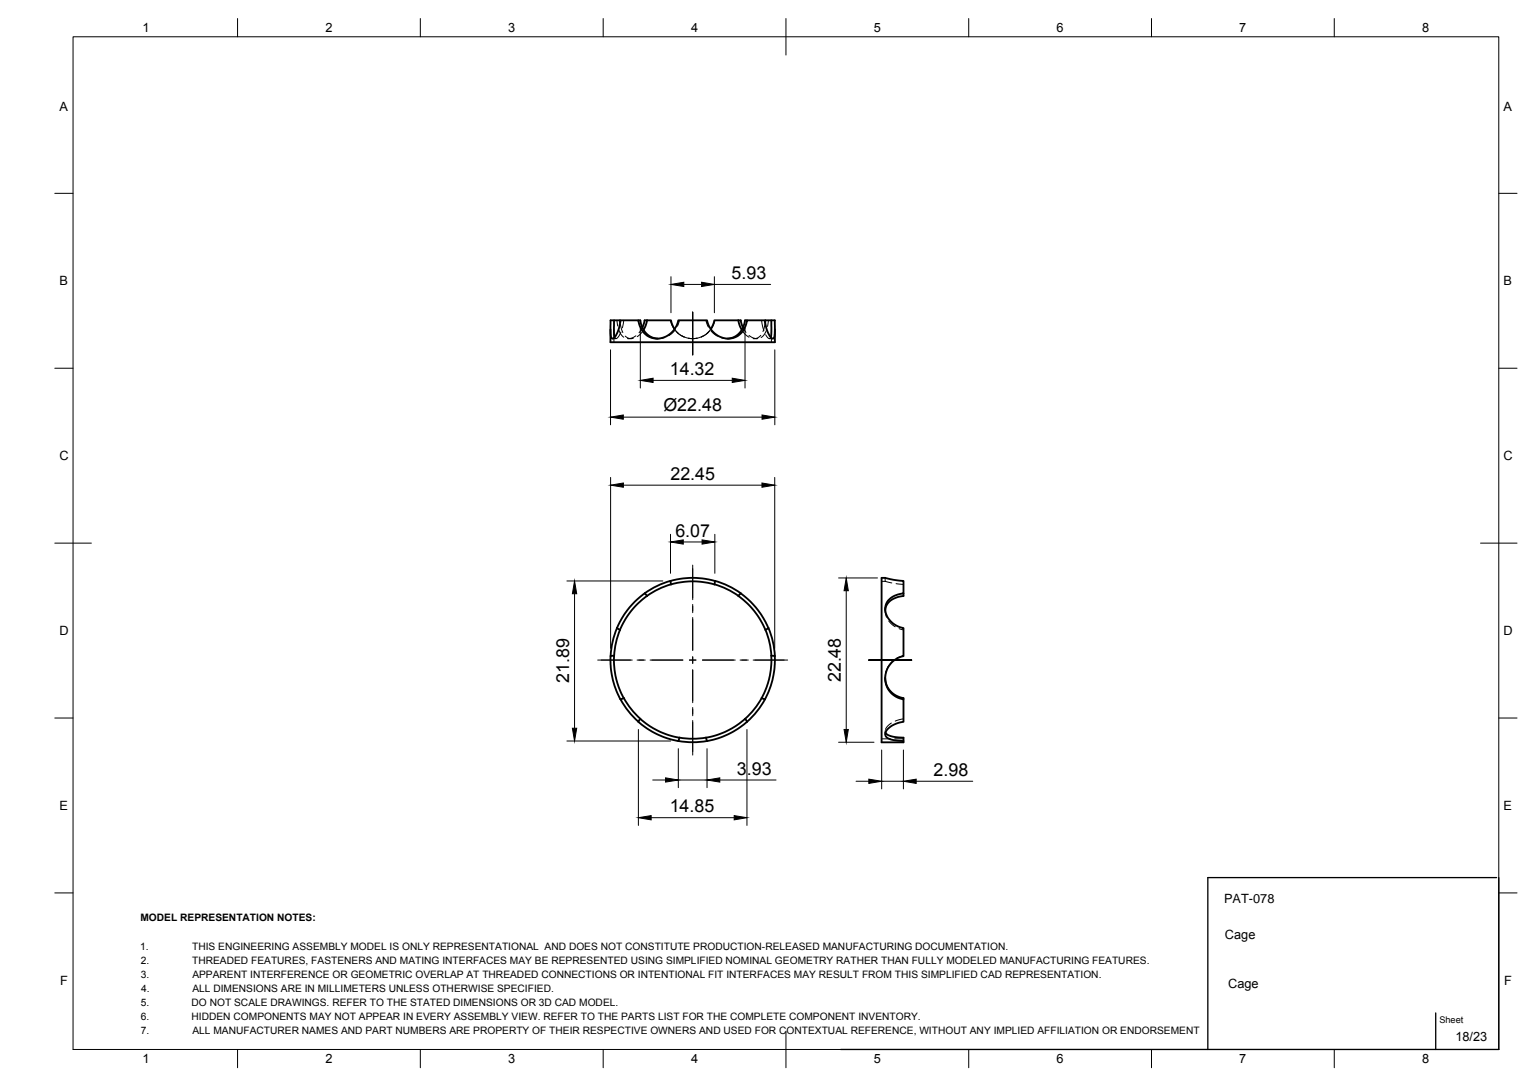
ISO-10303-21;
HEADER;
/* Generated by software containing ST-Developer
 * from STEP Tools, Inc. (www.steptools.com) 
 */

FILE_DESCRIPTION(
/* description */ ('Pedal-braked fixed caster'),
/* implementation_level */ '2;1');

FILE_NAME(
/* name */ 'Cage.step',
/* time_stamp */ '2026-10-28T03:26:52-07:00',
/* author */ (''),
/* organization */ (''),
/* preprocessor_version */ 'ST-DEVELOPER v20.2',
/* originating_system */ 'Autodesk Translation Framework v15.17.0.0',
/* authorisation */ '');

FILE_SCHEMA (('AUTOMOTIVE_DESIGN { 1 0 10303 214 3 1 1 }'));
ENDSEC;

DATA;
#10=MECHANICAL_DESIGN_GEOMETRIC_PRESENTATION_REPRESENTATION('',(#224),#5734);
#11=B_SPLINE_CURVE_WITH_KNOTS('',3,(#5151,#5152,#5153,#5154,#5155,#5156,
#5157,#5158,#5159,#5160,#5161,#5162,#5163,#5164,#5165,#5166,#5167,#5168,
#5169,#5170,#5171,#5172),.UNSPECIFIED.,.F.,.F.,(4,2,2,2,2,2,2,2,2,2,4),
(0.0591825211272536,0.157966726598481,0.236950089897721,0.315933453196962,
0.391576304923761,0.46721915665056,0.54286200837736,0.618504860104159,0.697488223403399,
0.77647158670264,0.875255792173867),.UNSPECIFIED.);
#12=B_SPLINE_CURVE_WITH_KNOTS('',3,(#5176,#5177,#5178,#5179,#5180,#5181,
#5182,#5183,#5184,#5185,#5186,#5187,#5188,#5189,#5190,#5191,#5192,#5193,
#5194,#5195,#5196,#5197),.UNSPECIFIED.,.F.,.F.,(4,2,2,2,2,2,2,2,2,2,4),
(0.0581119756758434,0.106553146291161,0.213106292582322,0.30849933801665,
0.386091982889075,0.4636846277615,0.541277272633925,0.61886991750635,0.714262962940678,
0.820816109231839,0.869257279847157),.UNSPECIFIED.);
#13=B_SPLINE_CURVE_WITH_KNOTS('',3,(#5203,#5204,#5205,#5206,#5207,#5208,
#5209,#5210,#5211,#5212,#5213,#5214,#5215,#5216,#5217,#5218,#5219,#5220,
#5221,#5222,#5223,#5224),.UNSPECIFIED.,.F.,.F.,(4,2,2,2,2,2,2,2,2,2,4),
(0.0581119756758434,0.106553146291161,0.213106292582322,0.30849933801665,
0.386091982889075,0.4636846277615,0.541277272633925,0.61886991750635,0.714262962940679,
0.820816109231839,0.869257279847157),.UNSPECIFIED.);
#14=B_SPLINE_CURVE_WITH_KNOTS('',3,(#5228,#5229,#5230,#5231,#5232,#5233,
#5234,#5235,#5236,#5237,#5238,#5239,#5240,#5241,#5242,#5243,#5244,#5245,
#5246,#5247,#5248,#5249),.UNSPECIFIED.,.F.,.F.,(4,2,2,2,2,2,2,2,2,2,4),
(0.0581119756758433,0.106553146291161,0.213106292582322,0.308499338016649,
0.386091982889075,0.4636846277615,0.541277272633925,0.61886991750635,0.714262962940678,
0.820816109231839,0.869257279847157),.UNSPECIFIED.);
#15=B_SPLINE_CURVE_WITH_KNOTS('',3,(#5258,#5259,#5260,#5261,#5262,#5263,
#5264,#5265,#5266,#5267,#5268,#5269,#5270,#5271,#5272,#5273,#5274,#5275,
#5276,#5277,#5278,#5279),.UNSPECIFIED.,.F.,.F.,(4,2,2,2,2,2,2,2,2,2,4),
(0.0581119756758433,0.106553146291161,0.213106292582322,0.30849933801665,
0.386091982889075,0.4636846277615,0.541277272633925,0.61886991750635,0.714262962940678,
0.820816109231839,0.869257279847157),.UNSPECIFIED.);
#16=B_SPLINE_CURVE_WITH_KNOTS('',3,(#5283,#5284,#5285,#5286,#5287,#5288,
#5289,#5290,#5291,#5292,#5293,#5294,#5295,#5296,#5297,#5298,#5299,#5300,
#5301,#5302,#5303,#5304),.UNSPECIFIED.,.F.,.F.,(4,2,2,2,2,2,2,2,2,2,4),
(0.0581119756758434,0.106553146291161,0.213106292582322,0.30849933801665,
0.386091982889075,0.4636846277615,0.541277272633925,0.61886991750635,0.714262962940678,
0.820816109231839,0.869257279847157),.UNSPECIFIED.);
#17=B_SPLINE_CURVE_WITH_KNOTS('',3,(#5308,#5309,#5310,#5311,#5312,#5313,
#5314,#5315,#5316,#5317,#5318,#5319,#5320,#5321,#5322,#5323,#5324,#5325,
#5326,#5327,#5328,#5329),.UNSPECIFIED.,.F.,.F.,(4,2,2,2,2,2,2,2,2,2,4),
(0.0581119756758434,0.106553146291161,0.213106292582322,0.30849933801665,
0.386091982889075,0.4636846277615,0.541277272633925,0.61886991750635,0.714262962940678,
0.820816109231839,0.869257279847157),.UNSPECIFIED.);
#18=B_SPLINE_CURVE_WITH_KNOTS('',3,(#5333,#5334,#5335,#5336,#5337,#5338,
#5339,#5340,#5341,#5342,#5343,#5344,#5345,#5346,#5347,#5348,#5349,#5350,
#5351,#5352,#5353,#5354),.UNSPECIFIED.,.F.,.F.,(4,2,2,2,2,2,2,2,2,2,4),
(0.0581119756758433,0.106553146291161,0.213106292582322,0.30849933801665,
0.386091982889075,0.4636846277615,0.541277272633925,0.61886991750635,0.714262962940678,
0.820816109231839,0.869257279847157),.UNSPECIFIED.);
#19=B_SPLINE_CURVE_WITH_KNOTS('',3,(#5362,#5363,#5364,#5365,#5366,#5367,
#5368,#5369,#5370,#5371,#5372,#5373,#5374,#5375,#5376,#5377,#5378,#5379,
#5380,#5381,#5382,#5383),.UNSPECIFIED.,.F.,.F.,(4,2,2,2,2,2,2,2,2,2,4),
(0.0591825211272536,0.157966726598481,0.236950089897721,0.315933453196962,
0.391576304923761,0.467219156650561,0.54286200837736,0.618504860104159,
0.697488223403399,0.77647158670264,0.875255792173867),.UNSPECIFIED.);
#20=B_SPLINE_CURVE_WITH_KNOTS('',3,(#5391,#5392,#5393,#5394,#5395,#5396,
#5397,#5398,#5399,#5400,#5401,#5402,#5403,#5404,#5405,#5406,#5407,#5408,
#5409,#5410,#5411,#5412),.UNSPECIFIED.,.F.,.F.,(4,2,2,2,2,2,2,2,2,2,4),
(0.0591825211272536,0.157966726598481,0.236950089897722,0.315933453196962,
0.391576304923761,0.467219156650561,0.54286200837736,0.618504860104159,
0.697488223403399,0.77647158670264,0.875255792173867),.UNSPECIFIED.);
#21=B_SPLINE_CURVE_WITH_KNOTS('',3,(#5422,#5423,#5424,#5425,#5426,#5427,
#5428,#5429,#5430,#5431,#5432,#5433,#5434,#5435,#5436,#5437,#5438,#5439,
#5440,#5441,#5442,#5443),.UNSPECIFIED.,.F.,.F.,(4,2,2,2,2,2,2,2,2,2,4),
(0.0591825211272536,0.157966726598481,0.236950089897721,0.315933453196962,
0.391576304923761,0.46721915665056,0.54286200837736,0.618504860104159,0.697488223403399,
0.77647158670264,0.875255792173867),.UNSPECIFIED.);
#22=B_SPLINE_CURVE_WITH_KNOTS('',3,(#5451,#5452,#5453,#5454,#5455,#5456,
#5457,#5458,#5459,#5460,#5461,#5462,#5463,#5464,#5465,#5466,#5467,#5468,
#5469,#5470,#5471,#5472),.UNSPECIFIED.,.F.,.F.,(4,2,2,2,2,2,2,2,2,2,4),
(0.0591825211272536,0.157966726598481,0.236950089897721,0.315933453196962,
0.391576304923761,0.46721915665056,0.542862008377359,0.618504860104159,
0.697488223403399,0.776471586702639,0.875255792173867),.UNSPECIFIED.);
#23=B_SPLINE_CURVE_WITH_KNOTS('',3,(#5480,#5481,#5482,#5483,#5484,#5485,
#5486,#5487,#5488,#5489,#5490,#5491,#5492,#5493,#5494,#5495,#5496,#5497,
#5498,#5499,#5500,#5501),.UNSPECIFIED.,.F.,.F.,(4,2,2,2,2,2,2,2,2,2,4),
(0.0591825211272536,0.157966726598481,0.236950089897721,0.315933453196962,
0.391576304923761,0.46721915665056,0.54286200837736,0.618504860104159,0.697488223403399,
0.77647158670264,0.875255792173867),.UNSPECIFIED.);
#24=B_SPLINE_CURVE_WITH_KNOTS('',3,(#5510,#5511,#5512,#5513,#5514,#5515,
#5516,#5517,#5518,#5519,#5520,#5521,#5522,#5523,#5524,#5525,#5526,#5527,
#5528,#5529,#5530,#5531),.UNSPECIFIED.,.F.,.F.,(4,2,2,2,2,2,2,2,2,2,4),
(0.0591825211272536,0.157966726598481,0.236950089897721,0.315933453196962,
0.391576304923761,0.46721915665056,0.542862008377359,0.618504860104159,
0.697488223403399,0.776471586702639,0.875255792173867),.UNSPECIFIED.);
#32=SPHERICAL_SURFACE('',#3444,0.309556);
#33=SPHERICAL_SURFACE('',#3460,0.309556);
#34=SPHERICAL_SURFACE('',#3465,0.309556);
#35=SPHERICAL_SURFACE('',#3471,0.309556);
#36=SPHERICAL_SURFACE('',#3476,0.309556);
#37=SPHERICAL_SURFACE('',#3481,0.309556);
#38=SPHERICAL_SURFACE('',#3489,0.309556);
#184=SHAPE_REPRESENTATION_RELATIONSHIP('SRR','None',#5824,#201);
#201=ADVANCED_BREP_SHAPE_REPRESENTATION('',(#247),#5728);
#224=STYLED_ITEM('',(#5984),#247);
#247=MANIFOLD_SOLID_BREP('Continuous crown cage',#3006);
#284=CYLINDRICAL_SURFACE('',#3447,1.123812);
#285=CYLINDRICAL_SURFACE('',#3483,1.076188);
#331=FACE_BOUND('',#837,.T.);
#426=CIRCLE('',#3445,0.303778037777585);
#427=CIRCLE('',#3446,0.303778037777585);
#428=CIRCLE('',#3448,1.123812);
#429=CIRCLE('',#3449,1.123812);
#430=CIRCLE('',#3450,1.123812);
#431=CIRCLE('',#3451,1.123812);
#432=CIRCLE('',#3452,1.123812);
#433=CIRCLE('',#3453,1.123812);
#434=CIRCLE('',#3454,1.123812);
#435=CIRCLE('',#3455,1.123812);
#436=CIRCLE('',#3456,1.123812);
#437=CIRCLE('',#3458,1.076188);
#438=CIRCLE('',#3459,0.303778037777585);
#439=CIRCLE('',#3461,0.303778037777585);
#440=CIRCLE('',#3463,1.076188);
#441=CIRCLE('',#3464,0.303778037777585);
#442=CIRCLE('',#3466,0.303778037777585);
#443=CIRCLE('',#3468,1.076188);
#444=CIRCLE('',#3469,1.076188);
#445=CIRCLE('',#3470,0.303778037777585);
#446=CIRCLE('',#3472,0.303778037777585);
#447=CIRCLE('',#3474,1.076188);
#448=CIRCLE('',#3475,0.303778037777585);
#449=CIRCLE('',#3477,0.303778037777585);
#450=CIRCLE('',#3479,1.076188);
#451=CIRCLE('',#3480,0.303778037777585);
#452=CIRCLE('',#3482,0.303778037777585);
#453=CIRCLE('',#3484,1.076188);
#454=CIRCLE('',#3485,1.076188);
#455=CIRCLE('',#3486,1.076188);
#456=CIRCLE('',#3488,0.303778037777585);
#457=CIRCLE('',#3490,0.303778037777585);
#607=FACE_OUTER_BOUND('',#821,.T.);
#608=FACE_OUTER_BOUND('',#822,.T.);
#609=FACE_OUTER_BOUND('',#823,.T.);
#610=FACE_OUTER_BOUND('',#824,.T.);
#611=FACE_OUTER_BOUND('',#825,.T.);
#612=FACE_OUTER_BOUND('',#826,.T.);
#613=FACE_OUTER_BOUND('',#827,.T.);
#614=FACE_OUTER_BOUND('',#828,.T.);
#615=FACE_OUTER_BOUND('',#829,.T.);
#616=FACE_OUTER_BOUND('',#830,.T.);
#617=FACE_OUTER_BOUND('',#831,.T.);
#618=FACE_OUTER_BOUND('',#832,.T.);
#619=FACE_OUTER_BOUND('',#833,.T.);
#620=FACE_OUTER_BOUND('',#834,.T.);
#621=FACE_OUTER_BOUND('',#835,.T.);
#622=FACE_OUTER_BOUND('',#836,.T.);
#623=FACE_OUTER_BOUND('',#838,.T.);
#821=EDGE_LOOP('',(#2484,#2485,#2486,#2487));
#822=EDGE_LOOP('',(#2488,#2489,#2490,#2491,#2492,#2493,#2494,#2495,#2496,
#2497,#2498,#2499,#2500,#2501,#2502,#2503,#2504,#2505));
#823=EDGE_LOOP('',(#2506,#2507,#2508,#2509));
#824=EDGE_LOOP('',(#2510,#2511,#2512,#2513));
#825=EDGE_LOOP('',(#2514,#2515,#2516,#2517));
#826=EDGE_LOOP('',(#2518,#2519,#2520,#2521));
#827=EDGE_LOOP('',(#2522,#2523,#2524,#2525,#2526,#2527));
#828=EDGE_LOOP('',(#2528,#2529,#2530,#2531));
#829=EDGE_LOOP('',(#2532,#2533,#2534,#2535));
#830=EDGE_LOOP('',(#2536,#2537,#2538,#2539));
#831=EDGE_LOOP('',(#2540,#2541,#2542,#2543));
#832=EDGE_LOOP('',(#2544,#2545,#2546,#2547));
#833=EDGE_LOOP('',(#2548,#2549,#2550,#2551,#2552,#2553,#2554,#2555,#2556,
#2557,#2558,#2559,#2560,#2561,#2562,#2563,#2564,#2565));
#834=EDGE_LOOP('',(#2566,#2567,#2568,#2569));
#835=EDGE_LOOP('',(#2570,#2571,#2572,#2573));
#836=EDGE_LOOP('',(#2574));
#837=EDGE_LOOP('',(#2575));
#838=EDGE_LOOP('',(#2576,#2577,#2578,#2579));
#1045=LINE('',#5253,#1257);
#1046=LINE('',#5506,#1258);
#1257=VECTOR('',#4231,1.123812);
#1258=VECTOR('',#4300,1.076188);
#1488=VERTEX_POINT('',#5149);
#1489=VERTEX_POINT('',#5150);
#1490=VERTEX_POINT('',#5173);
#1491=VERTEX_POINT('',#5175);
#1492=VERTEX_POINT('',#5200);
#1493=VERTEX_POINT('',#5202);
#1494=VERTEX_POINT('',#5225);
#1495=VERTEX_POINT('',#5227);
#1496=VERTEX_POINT('',#5250);
#1497=VERTEX_POINT('',#5252);
#1498=VERTEX_POINT('',#5255);
#1499=VERTEX_POINT('',#5257);
#1500=VERTEX_POINT('',#5280);
#1501=VERTEX_POINT('',#5282);
#1502=VERTEX_POINT('',#5305);
#1503=VERTEX_POINT('',#5307);
#1504=VERTEX_POINT('',#5330);
#1505=VERTEX_POINT('',#5332);
#1506=VERTEX_POINT('',#5357);
#1507=VERTEX_POINT('',#5361);
#1508=VERTEX_POINT('',#5386);
#1509=VERTEX_POINT('',#5390);
#1510=VERTEX_POINT('',#5415);
#1511=VERTEX_POINT('',#5417);
#1512=VERTEX_POINT('',#5421);
#1513=VERTEX_POINT('',#5446);
#1514=VERTEX_POINT('',#5450);
#1515=VERTEX_POINT('',#5475);
#1516=VERTEX_POINT('',#5479);
#1517=VERTEX_POINT('',#5504);
#1518=VERTEX_POINT('',#5507);
#1519=VERTEX_POINT('',#5509);
#1832=EDGE_CURVE('',#1488,#1489,#11,.T.);
#1833=EDGE_CURVE('',#1490,#1488,#426,.T.);
#1834=EDGE_CURVE('',#1491,#1490,#12,.T.);
#1835=EDGE_CURVE('',#1489,#1491,#427,.T.);
#1836=EDGE_CURVE('',#1492,#1490,#428,.T.);
#1837=EDGE_CURVE('',#1492,#1493,#13,.T.);
#1838=EDGE_CURVE('',#1494,#1493,#429,.T.);
#1839=EDGE_CURVE('',#1494,#1495,#14,.T.);
#1840=EDGE_CURVE('',#1496,#1495,#430,.T.);
#1841=EDGE_CURVE('',#1496,#1497,#1045,.T.);
#1842=EDGE_CURVE('',#1497,#1497,#431,.T.);
#1843=EDGE_CURVE('',#1498,#1496,#432,.T.);
#1844=EDGE_CURVE('',#1498,#1499,#15,.T.);
#1845=EDGE_CURVE('',#1500,#1499,#433,.T.);
#1846=EDGE_CURVE('',#1500,#1501,#16,.T.);
#1847=EDGE_CURVE('',#1502,#1501,#434,.T.);
#1848=EDGE_CURVE('',#1502,#1503,#17,.T.);
#1849=EDGE_CURVE('',#1504,#1503,#435,.T.);
#1850=EDGE_CURVE('',#1504,#1505,#18,.T.);
#1851=EDGE_CURVE('',#1491,#1505,#436,.T.);
#1852=EDGE_CURVE('',#1488,#1506,#437,.T.);
#1853=EDGE_CURVE('',#1506,#1492,#438,.T.);
#1854=EDGE_CURVE('',#1507,#1506,#19,.T.);
#1855=EDGE_CURVE('',#1493,#1507,#439,.T.);
#1856=EDGE_CURVE('',#1507,#1508,#440,.T.);
#1857=EDGE_CURVE('',#1508,#1494,#441,.T.);
#1858=EDGE_CURVE('',#1509,#1508,#20,.T.);
#1859=EDGE_CURVE('',#1495,#1509,#442,.T.);
#1860=EDGE_CURVE('',#1509,#1510,#443,.T.);
#1861=EDGE_CURVE('',#1510,#1511,#444,.T.);
#1862=EDGE_CURVE('',#1511,#1498,#445,.T.);
#1863=EDGE_CURVE('',#1512,#1511,#21,.T.);
#1864=EDGE_CURVE('',#1499,#1512,#446,.T.);
#1865=EDGE_CURVE('',#1512,#1513,#447,.T.);
#1866=EDGE_CURVE('',#1513,#1500,#448,.T.);
#1867=EDGE_CURVE('',#1514,#1513,#22,.T.);
#1868=EDGE_CURVE('',#1501,#1514,#449,.T.);
#1869=EDGE_CURVE('',#1514,#1515,#450,.T.);
#1870=EDGE_CURVE('',#1515,#1502,#451,.T.);
#1871=EDGE_CURVE('',#1516,#1515,#23,.T.);
#1872=EDGE_CURVE('',#1503,#1516,#452,.T.);
#1873=EDGE_CURVE('',#1517,#1517,#453,.T.);
#1874=EDGE_CURVE('',#1517,#1510,#1046,.T.);
#1875=EDGE_CURVE('',#1518,#1489,#454,.T.);
#1876=EDGE_CURVE('',#1518,#1519,#24,.T.);
#1877=EDGE_CURVE('',#1516,#1519,#455,.T.);
#1878=EDGE_CURVE('',#1505,#1518,#456,.T.);
#1879=EDGE_CURVE('',#1519,#1504,#457,.T.);
#2484=ORIENTED_EDGE('',*,*,#1832,.F.);
#2485=ORIENTED_EDGE('',*,*,#1833,.F.);
#2486=ORIENTED_EDGE('',*,*,#1834,.F.);
#2487=ORIENTED_EDGE('',*,*,#1835,.F.);
#2488=ORIENTED_EDGE('',*,*,#1834,.T.);
#2489=ORIENTED_EDGE('',*,*,#1836,.F.);
#2490=ORIENTED_EDGE('',*,*,#1837,.T.);
#2491=ORIENTED_EDGE('',*,*,#1838,.F.);
#2492=ORIENTED_EDGE('',*,*,#1839,.T.);
#2493=ORIENTED_EDGE('',*,*,#1840,.F.);
#2494=ORIENTED_EDGE('',*,*,#1841,.T.);
#2495=ORIENTED_EDGE('',*,*,#1842,.F.);
#2496=ORIENTED_EDGE('',*,*,#1841,.F.);
#2497=ORIENTED_EDGE('',*,*,#1843,.F.);
#2498=ORIENTED_EDGE('',*,*,#1844,.T.);
#2499=ORIENTED_EDGE('',*,*,#1845,.F.);
#2500=ORIENTED_EDGE('',*,*,#1846,.T.);
#2501=ORIENTED_EDGE('',*,*,#1847,.F.);
#2502=ORIENTED_EDGE('',*,*,#1848,.T.);
#2503=ORIENTED_EDGE('',*,*,#1849,.F.);
#2504=ORIENTED_EDGE('',*,*,#1850,.T.);
#2505=ORIENTED_EDGE('',*,*,#1851,.F.);
#2506=ORIENTED_EDGE('',*,*,#1833,.T.);
#2507=ORIENTED_EDGE('',*,*,#1852,.T.);
#2508=ORIENTED_EDGE('',*,*,#1853,.T.);
#2509=ORIENTED_EDGE('',*,*,#1836,.T.);
#2510=ORIENTED_EDGE('',*,*,#1854,.F.);
#2511=ORIENTED_EDGE('',*,*,#1855,.F.);
#2512=ORIENTED_EDGE('',*,*,#1837,.F.);
#2513=ORIENTED_EDGE('',*,*,#1853,.F.);
#2514=ORIENTED_EDGE('',*,*,#1855,.T.);
#2515=ORIENTED_EDGE('',*,*,#1856,.T.);
#2516=ORIENTED_EDGE('',*,*,#1857,.T.);
#2517=ORIENTED_EDGE('',*,*,#1838,.T.);
#2518=ORIENTED_EDGE('',*,*,#1858,.F.);
#2519=ORIENTED_EDGE('',*,*,#1859,.F.);
#2520=ORIENTED_EDGE('',*,*,#1839,.F.);
#2521=ORIENTED_EDGE('',*,*,#1857,.F.);
#2522=ORIENTED_EDGE('',*,*,#1859,.T.);
#2523=ORIENTED_EDGE('',*,*,#1860,.T.);
#2524=ORIENTED_EDGE('',*,*,#1861,.T.);
#2525=ORIENTED_EDGE('',*,*,#1862,.T.);
#2526=ORIENTED_EDGE('',*,*,#1843,.T.);
#2527=ORIENTED_EDGE('',*,*,#1840,.T.);
#2528=ORIENTED_EDGE('',*,*,#1863,.F.);
#2529=ORIENTED_EDGE('',*,*,#1864,.F.);
#2530=ORIENTED_EDGE('',*,*,#1844,.F.);
#2531=ORIENTED_EDGE('',*,*,#1862,.F.);
#2532=ORIENTED_EDGE('',*,*,#1864,.T.);
#2533=ORIENTED_EDGE('',*,*,#1865,.T.);
#2534=ORIENTED_EDGE('',*,*,#1866,.T.);
#2535=ORIENTED_EDGE('',*,*,#1845,.T.);
#2536=ORIENTED_EDGE('',*,*,#1867,.F.);
#2537=ORIENTED_EDGE('',*,*,#1868,.F.);
#2538=ORIENTED_EDGE('',*,*,#1846,.F.);
#2539=ORIENTED_EDGE('',*,*,#1866,.F.);
#2540=ORIENTED_EDGE('',*,*,#1868,.T.);
#2541=ORIENTED_EDGE('',*,*,#1869,.T.);
#2542=ORIENTED_EDGE('',*,*,#1870,.T.);
#2543=ORIENTED_EDGE('',*,*,#1847,.T.);
#2544=ORIENTED_EDGE('',*,*,#1848,.F.);
#2545=ORIENTED_EDGE('',*,*,#1870,.F.);
#2546=ORIENTED_EDGE('',*,*,#1871,.F.);
#2547=ORIENTED_EDGE('',*,*,#1872,.F.);
#2548=ORIENTED_EDGE('',*,*,#1873,.F.);
#2549=ORIENTED_EDGE('',*,*,#1874,.T.);
#2550=ORIENTED_EDGE('',*,*,#1860,.F.);
#2551=ORIENTED_EDGE('',*,*,#1858,.T.);
#2552=ORIENTED_EDGE('',*,*,#1856,.F.);
#2553=ORIENTED_EDGE('',*,*,#1854,.T.);
#2554=ORIENTED_EDGE('',*,*,#1852,.F.);
#2555=ORIENTED_EDGE('',*,*,#1832,.T.);
#2556=ORIENTED_EDGE('',*,*,#1875,.F.);
#2557=ORIENTED_EDGE('',*,*,#1876,.T.);
#2558=ORIENTED_EDGE('',*,*,#1877,.F.);
#2559=ORIENTED_EDGE('',*,*,#1871,.T.);
#2560=ORIENTED_EDGE('',*,*,#1869,.F.);
#2561=ORIENTED_EDGE('',*,*,#1867,.T.);
#2562=ORIENTED_EDGE('',*,*,#1865,.F.);
#2563=ORIENTED_EDGE('',*,*,#1863,.T.);
#2564=ORIENTED_EDGE('',*,*,#1861,.F.);
#2565=ORIENTED_EDGE('',*,*,#1874,.F.);
#2566=ORIENTED_EDGE('',*,*,#1835,.T.);
#2567=ORIENTED_EDGE('',*,*,#1851,.T.);
#2568=ORIENTED_EDGE('',*,*,#1878,.T.);
#2569=ORIENTED_EDGE('',*,*,#1875,.T.);
#2570=ORIENTED_EDGE('',*,*,#1850,.F.);
#2571=ORIENTED_EDGE('',*,*,#1879,.F.);
#2572=ORIENTED_EDGE('',*,*,#1876,.F.);
#2573=ORIENTED_EDGE('',*,*,#1878,.F.);
#2574=ORIENTED_EDGE('',*,*,#1842,.T.);
#2575=ORIENTED_EDGE('',*,*,#1873,.T.);
#2576=ORIENTED_EDGE('',*,*,#1872,.T.);
#2577=ORIENTED_EDGE('',*,*,#1877,.T.);
#2578=ORIENTED_EDGE('',*,*,#1879,.T.);
#2579=ORIENTED_EDGE('',*,*,#1849,.T.);
#2780=PLANE('',#3457);
#2781=PLANE('',#3462);
#2782=PLANE('',#3467);
#2783=PLANE('',#3473);
#2784=PLANE('',#3478);
#2785=PLANE('',#3487);
#2786=PLANE('',#3491);
#2787=PLANE('',#3492);
#2940=ADVANCED_FACE('',(#607),#32,.F.);
#2941=ADVANCED_FACE('',(#608),#284,.T.);
#2942=ADVANCED_FACE('',(#609),#2780,.T.);
#2943=ADVANCED_FACE('',(#610),#33,.F.);
#2944=ADVANCED_FACE('',(#611),#2781,.T.);
#2945=ADVANCED_FACE('',(#612),#34,.F.);
#2946=ADVANCED_FACE('',(#613),#2782,.T.);
#2947=ADVANCED_FACE('',(#614),#35,.F.);
#2948=ADVANCED_FACE('',(#615),#2783,.T.);
#2949=ADVANCED_FACE('',(#616),#36,.F.);
#2950=ADVANCED_FACE('',(#617),#2784,.T.);
#2951=ADVANCED_FACE('',(#618),#37,.F.);
#2952=ADVANCED_FACE('',(#619),#285,.F.);
#2953=ADVANCED_FACE('',(#620),#2785,.T.);
#2954=ADVANCED_FACE('',(#621),#38,.F.);
#2955=ADVANCED_FACE('',(#622,#331),#2786,.T.);
#2956=ADVANCED_FACE('',(#623),#2787,.T.);
#3006=CLOSED_SHELL('',(#2940,#2941,#2942,#2943,#2944,#2945,#2946,#2947,
#2948,#2949,#2950,#2951,#2952,#2953,#2954,#2955,#2956));
#3443=AXIS2_PLACEMENT_3D('',#5147,#4215,#4216);
#3444=AXIS2_PLACEMENT_3D('',#5148,#4217,#4218);
#3445=AXIS2_PLACEMENT_3D('',#5174,#4219,#4220);
#3446=AXIS2_PLACEMENT_3D('',#5198,#4221,#4222);
#3447=AXIS2_PLACEMENT_3D('',#5199,#4223,#4224);
#3448=AXIS2_PLACEMENT_3D('',#5201,#4225,#4226);
#3449=AXIS2_PLACEMENT_3D('',#5226,#4227,#4228);
#3450=AXIS2_PLACEMENT_3D('',#5251,#4229,#4230);
#3451=AXIS2_PLACEMENT_3D('',#5254,#4232,#4233);
#3452=AXIS2_PLACEMENT_3D('',#5256,#4234,#4235);
#3453=AXIS2_PLACEMENT_3D('',#5281,#4236,#4237);
#3454=AXIS2_PLACEMENT_3D('',#5306,#4238,#4239);
#3455=AXIS2_PLACEMENT_3D('',#5331,#4240,#4241);
#3456=AXIS2_PLACEMENT_3D('',#5355,#4242,#4243);
#3457=AXIS2_PLACEMENT_3D('',#5356,#4244,#4245);
#3458=AXIS2_PLACEMENT_3D('',#5358,#4246,#4247);
#3459=AXIS2_PLACEMENT_3D('',#5359,#4248,#4249);
#3460=AXIS2_PLACEMENT_3D('',#5360,#4250,#4251);
#3461=AXIS2_PLACEMENT_3D('',#5384,#4252,#4253);
#3462=AXIS2_PLACEMENT_3D('',#5385,#4254,#4255);
#3463=AXIS2_PLACEMENT_3D('',#5387,#4256,#4257);
#3464=AXIS2_PLACEMENT_3D('',#5388,#4258,#4259);
#3465=AXIS2_PLACEMENT_3D('',#5389,#4260,#4261);
#3466=AXIS2_PLACEMENT_3D('',#5413,#4262,#4263);
#3467=AXIS2_PLACEMENT_3D('',#5414,#4264,#4265);
#3468=AXIS2_PLACEMENT_3D('',#5416,#4266,#4267);
#3469=AXIS2_PLACEMENT_3D('',#5418,#4268,#4269);
#3470=AXIS2_PLACEMENT_3D('',#5419,#4270,#4271);
#3471=AXIS2_PLACEMENT_3D('',#5420,#4272,#4273);
#3472=AXIS2_PLACEMENT_3D('',#5444,#4274,#4275);
#3473=AXIS2_PLACEMENT_3D('',#5445,#4276,#4277);
#3474=AXIS2_PLACEMENT_3D('',#5447,#4278,#4279);
#3475=AXIS2_PLACEMENT_3D('',#5448,#4280,#4281);
#3476=AXIS2_PLACEMENT_3D('',#5449,#4282,#4283);
#3477=AXIS2_PLACEMENT_3D('',#5473,#4284,#4285);
#3478=AXIS2_PLACEMENT_3D('',#5474,#4286,#4287);
#3479=AXIS2_PLACEMENT_3D('',#5476,#4288,#4289);
#3480=AXIS2_PLACEMENT_3D('',#5477,#4290,#4291);
#3481=AXIS2_PLACEMENT_3D('',#5478,#4292,#4293);
#3482=AXIS2_PLACEMENT_3D('',#5502,#4294,#4295);
#3483=AXIS2_PLACEMENT_3D('',#5503,#4296,#4297);
#3484=AXIS2_PLACEMENT_3D('',#5505,#4298,#4299);
#3485=AXIS2_PLACEMENT_3D('',#5508,#4301,#4302);
#3486=AXIS2_PLACEMENT_3D('',#5532,#4303,#4304);
#3487=AXIS2_PLACEMENT_3D('',#5533,#4305,#4306);
#3488=AXIS2_PLACEMENT_3D('',#5534,#4307,#4308);
#3489=AXIS2_PLACEMENT_3D('',#5535,#4309,#4310);
#3490=AXIS2_PLACEMENT_3D('',#5536,#4311,#4312);
#3491=AXIS2_PLACEMENT_3D('',#5537,#4313,#4314);
#3492=AXIS2_PLACEMENT_3D('',#5538,#4315,#4316);
#4215=DIRECTION('axis',(0.,0.,1.));
#4216=DIRECTION('refdir',(1.,0.,0.));
#4217=DIRECTION('center_axis',(0.,0.,1.));
#4218=DIRECTION('ref_axis',(1.,0.,0.));
#4219=DIRECTION('center_axis',(0.,-1.,0.));
#4220=DIRECTION('ref_axis',(0.,0.,-1.));
#4221=DIRECTION('center_axis',(0.,-1.,0.));
#4222=DIRECTION('ref_axis',(0.,0.,-1.));
#4223=DIRECTION('center_axis',(0.,1.,0.));
#4224=DIRECTION('ref_axis',(1.,0.,0.));
#4225=DIRECTION('center_axis',(0.,1.,0.));
#4226=DIRECTION('ref_axis',(1.,0.,0.));
#4227=DIRECTION('center_axis',(0.,1.,0.));
#4228=DIRECTION('ref_axis',(1.,0.,0.));
#4229=DIRECTION('center_axis',(0.,1.,0.));
#4230=DIRECTION('ref_axis',(1.,0.,0.));
#4231=DIRECTION('',(0.,-1.,0.));
#4232=DIRECTION('center_axis',(0.,-1.,0.));
#4233=DIRECTION('ref_axis',(1.,0.,0.));
#4234=DIRECTION('center_axis',(0.,1.,0.));
#4235=DIRECTION('ref_axis',(1.,0.,0.));
#4236=DIRECTION('center_axis',(0.,1.,0.));
#4237=DIRECTION('ref_axis',(1.,0.,0.));
#4238=DIRECTION('center_axis',(0.,1.,0.));
#4239=DIRECTION('ref_axis',(1.,0.,0.));
#4240=DIRECTION('center_axis',(0.,1.,0.));
#4241=DIRECTION('ref_axis',(1.,0.,0.));
#4242=DIRECTION('center_axis',(0.,1.,0.));
#4243=DIRECTION('ref_axis',(1.,0.,0.));
#4244=DIRECTION('center_axis',(0.,1.,0.));
#4245=DIRECTION('ref_axis',(1.,0.,0.));
#4246=DIRECTION('center_axis',(0.,-1.,0.));
#4247=DIRECTION('ref_axis',(1.,0.,0.));
#4248=DIRECTION('center_axis',(0.,-1.,0.));
#4249=DIRECTION('ref_axis',(0.,0.,-1.));
#4250=DIRECTION('center_axis',(8.96625347776458E-17,0.,1.));
#4251=DIRECTION('ref_axis',(1.,0.,0.));
#4252=DIRECTION('center_axis',(0.,-1.,0.));
#4253=DIRECTION('ref_axis',(0.,0.,-1.));
#4254=DIRECTION('center_axis',(0.,1.,0.));
#4255=DIRECTION('ref_axis',(1.,0.,0.));
#4256=DIRECTION('center_axis',(0.,-1.,0.));
#4257=DIRECTION('ref_axis',(1.,0.,0.));
#4258=DIRECTION('center_axis',(0.,-1.,0.));
#4259=DIRECTION('ref_axis',(0.,0.,-1.));
#4260=DIRECTION('center_axis',(0.,0.,1.));
#4261=DIRECTION('ref_axis',(1.,0.,0.));
#4262=DIRECTION('center_axis',(0.,-1.,0.));
#4263=DIRECTION('ref_axis',(0.,0.,-1.));
#4264=DIRECTION('center_axis',(0.,1.,0.));
#4265=DIRECTION('ref_axis',(1.,0.,0.));
#4266=DIRECTION('center_axis',(0.,-1.,0.));
#4267=DIRECTION('ref_axis',(1.,0.,0.));
#4268=DIRECTION('center_axis',(0.,-1.,0.));
#4269=DIRECTION('ref_axis',(1.,0.,0.));
#4270=DIRECTION('center_axis',(0.,-1.,0.));
#4271=DIRECTION('ref_axis',(0.,0.,-1.));
#4272=DIRECTION('center_axis',(0.,0.,1.));
#4273=DIRECTION('ref_axis',(1.,0.,0.));
#4274=DIRECTION('center_axis',(0.,-1.,0.));
#4275=DIRECTION('ref_axis',(0.,0.,-1.));
#4276=DIRECTION('center_axis',(0.,1.,0.));
#4277=DIRECTION('ref_axis',(1.,0.,0.));
#4278=DIRECTION('center_axis',(0.,-1.,0.));
#4279=DIRECTION('ref_axis',(1.,0.,0.));
#4280=DIRECTION('center_axis',(0.,-1.,0.));
#4281=DIRECTION('ref_axis',(0.,0.,-1.));
#4282=DIRECTION('center_axis',(8.96625347776458E-17,0.,1.));
#4283=DIRECTION('ref_axis',(1.,0.,0.));
#4284=DIRECTION('center_axis',(0.,-1.,0.));
#4285=DIRECTION('ref_axis',(0.,0.,-1.));
#4286=DIRECTION('center_axis',(0.,1.,0.));
#4287=DIRECTION('ref_axis',(1.,0.,0.));
#4288=DIRECTION('center_axis',(0.,-1.,0.));
#4289=DIRECTION('ref_axis',(1.,0.,0.));
#4290=DIRECTION('center_axis',(0.,-1.,0.));
#4291=DIRECTION('ref_axis',(0.,0.,-1.));
#4292=DIRECTION('center_axis',(0.,0.,1.));
#4293=DIRECTION('ref_axis',(1.,0.,0.));
#4294=DIRECTION('center_axis',(0.,-1.,0.));
#4295=DIRECTION('ref_axis',(0.,0.,-1.));
#4296=DIRECTION('center_axis',(0.,1.,0.));
#4297=DIRECTION('ref_axis',(1.,0.,0.));
#4298=DIRECTION('center_axis',(0.,1.,0.));
#4299=DIRECTION('ref_axis',(1.,0.,0.));
#4300=DIRECTION('',(0.,1.,0.));
#4301=DIRECTION('center_axis',(0.,-1.,0.));
#4302=DIRECTION('ref_axis',(1.,0.,0.));
#4303=DIRECTION('center_axis',(0.,-1.,0.));
#4304=DIRECTION('ref_axis',(1.,0.,0.));
#4305=DIRECTION('center_axis',(0.,1.,0.));
#4306=DIRECTION('ref_axis',(1.,0.,0.));
#4307=DIRECTION('center_axis',(0.,-1.,0.));
#4308=DIRECTION('ref_axis',(0.,0.,-1.));
#4309=DIRECTION('center_axis',(0.,0.,1.));
#4310=DIRECTION('ref_axis',(1.,0.,0.));
#4311=DIRECTION('center_axis',(0.,-1.,0.));
#4312=DIRECTION('ref_axis',(0.,0.,-1.));
#4313=DIRECTION('center_axis',(0.,-1.,0.));
#4314=DIRECTION('ref_axis',(-1.,0.,0.));
#4315=DIRECTION('center_axis',(0.,1.,0.));
#4316=DIRECTION('ref_axis',(1.,0.,0.));
#5147=CARTESIAN_POINT('',(0.,0.,0.));
#5148=CARTESIAN_POINT('Origin',(0.685838782044607,0.,0.860014630714833));
#5149=CARTESIAN_POINT('',(0.413083465285518,-0.05953,0.993751811093549));
#5150=CARTESIAN_POINT('',(0.876916659919095,-0.05953,0.623857181492959));
#5151=CARTESIAN_POINT('Ctrl Pts',(0.413083465285518,-0.05953,0.993751811093549));
#5152=CARTESIAN_POINT('Ctrl Pts',(0.419070565453383,-0.0925528133349865,
0.991263089003441));
#5153=CARTESIAN_POINT('Ctrl Pts',(0.430199341854858,-0.124911173756694,
0.986608710139579));
#5154=CARTESIAN_POINT('Ctrl Pts',(0.457978755888596,-0.177924977804098,
0.973971221090534));
#5155=CARTESIAN_POINT('Ctrl Pts',(0.473077587363685,-0.199697230012983,
0.966820759530997));
#5156=CARTESIAN_POINT('Ctrl Pts',(0.507057380724533,-0.237895043532788,
0.949440676105255));
#5157=CARTESIAN_POINT('Ctrl Pts',(0.525933334162555,-0.254319232363049,
0.939198248544428));
#5158=CARTESIAN_POINT('Ctrl Pts',(0.564362943424238,-0.28018331644634,0.916597376014514));
#5159=CARTESIAN_POINT('Ctrl Pts',(0.585840553788742,-0.29104845371857,0.903141581680914));
#5160=CARTESIAN_POINT('Ctrl Pts',(0.629305439856167,-0.30527573347708,0.873412008702649));
#5161=CARTESIAN_POINT('Ctrl Pts',(0.651278921914856,-0.308638795020976,
0.857118508332695));
#5162=CARTESIAN_POINT('Ctrl Pts',(0.690705563850638,-0.308638795020976,
0.825676810575914));
#5163=CARTESIAN_POINT('Ctrl Pts',(0.711480111898423,-0.30527573347708,0.807879894508811));
#5164=CARTESIAN_POINT('Ctrl Pts',(0.750136149454208,-0.29104845371857,0.772120216227122));
#5165=CARTESIAN_POINT('Ctrl Pts',(0.768033796848072,-0.28018331644634,0.754175290318038));
#5166=CARTESIAN_POINT('Ctrl Pts',(0.798619410861634,-0.254319232363049,
0.721738358858166));
#5167=CARTESIAN_POINT('Ctrl Pts',(0.812805334167529,-0.237895043532788,
0.705614819529209));
#5168=CARTESIAN_POINT('Ctrl Pts',(0.837310877969633,-0.199697230012983,
0.676354402927683));
#5169=CARTESIAN_POINT('Ctrl Pts',(0.847641868610495,-0.177924977804098,
0.663225258065736));
#5170=CARTESIAN_POINT('Ctrl Pts',(0.866144010579847,-0.124911173756694,
0.638954437806245));
#5171=CARTESIAN_POINT('Ctrl Pts',(0.873158080166742,-0.0925528133349865,
0.62914037979579));
#5172=CARTESIAN_POINT('Ctrl Pts',(0.876916659919095,-0.05953,0.623857181492959));
#5173=CARTESIAN_POINT('',(0.437601487681057,-0.05953,1.03511272300331));
#5174=CARTESIAN_POINT('Origin',(0.685838782044607,-0.05953,0.860014630714833));
#5175=CARTESIAN_POINT('',(0.911784794170997,-0.05953,0.656964154625313));
#5176=CARTESIAN_POINT('Ctrl Pts',(0.911784794170998,-0.0595300000000001,
0.656964154625312));
#5177=CARTESIAN_POINT('Ctrl Pts',(0.909827729890942,-0.0762225747374255,
0.659680317203144));
#5178=CARTESIAN_POINT('Ctrl Pts',(0.907004864562642,-0.0928409665394228,
0.663576540841106));
#5179=CARTESIAN_POINT('Ctrl Pts',(0.895234408667242,-0.144299303100741,
0.679480524217551));
#5180=CARTESIAN_POINT('Ctrl Pts',(0.882797231409153,-0.177024326825049,
0.695831250979106));
#5181=CARTESIAN_POINT('Ctrl Pts',(0.854332839576145,-0.227269801620064,
0.73042219438957));
#5182=CARTESIAN_POINT('Ctrl Pts',(0.834863020612702,-0.251265615809407,
0.752807465209441));
#5183=CARTESIAN_POINT('Ctrl Pts',(0.800439809856111,-0.279889827963178,
0.789147407129766));
#5184=CARTESIAN_POINT('Ctrl Pts',(0.781998747691871,-0.290879136862659,
0.80756613568454));
#5185=CARTESIAN_POINT('Ctrl Pts',(0.742239891936898,-0.305251990234487,
0.844254137480382));
#5186=CARTESIAN_POINT('Ctrl Pts',(0.720906778729541,-0.308638795020976,
0.862505527716294));
#5187=CARTESIAN_POINT('Ctrl Pts',(0.680463863683392,-0.308638795020976,
0.894757676234429));
#5188=CARTESIAN_POINT('Ctrl Pts',(0.657923009631182,-0.305251990234488,
0.91149460735272));
#5189=CARTESIAN_POINT('Ctrl Pts',(0.613307674922609,-0.290879136862659,
0.942092777160053));
#5190=CARTESIAN_POINT('Ctrl Pts',(0.591247219971725,-0.279889827963178,
0.955972930713954));
#5191=CARTESIAN_POINT('Ctrl Pts',(0.548158511259202,-0.251265615809407,
0.981446681891443));
#5192=CARTESIAN_POINT('Ctrl Pts',(0.522002043615455,-0.227269801620063,
0.995447160474328));
#5193=CARTESIAN_POINT('Ctrl Pts',(0.481944444320713,-0.177024326825049,
1.01550068154148));
#5194=CARTESIAN_POINT('Ctrl Pts',(0.463236132117164,-0.14429930310074,1.0239876538093));
#5195=CARTESIAN_POINT('Ctrl Pts',(0.445111721969657,-0.0928409665394226,
1.03192403056628));
#5196=CARTESIAN_POINT('Ctrl Pts',(0.440685038163619,-0.0762225747374254,
1.03380912944435));
#5197=CARTESIAN_POINT('Ctrl Pts',(0.437601487681056,-0.05953,1.03511272300331));
#5198=CARTESIAN_POINT('Origin',(0.685838782044607,-0.05953,0.860014630714833));
#5199=CARTESIAN_POINT('Origin',(0.,-0.208355,0.));
#5200=CARTESIAN_POINT('',(0.0548532617164168,-0.05953,1.12247250791415));
#5201=CARTESIAN_POINT('Origin',(0.,-0.05953,0.));
#5202=CARTESIAN_POINT('',(-0.536443649899848,-0.05953,0.987512846410683));
#5203=CARTESIAN_POINT('Ctrl Pts',(0.0548532617164173,-0.0595300000000001,
1.12247250791414));
#5204=CARTESIAN_POINT('Ctrl Pts',(0.05150947068137,-0.0762225747374254,
1.12263591311425));
#5205=CARTESIAN_POINT('Ctrl Pts',(0.0467032526342597,-0.0928409665394227,
1.12285816383385));
#5206=CARTESIAN_POINT('Ctrl Pts',(0.0269302585198975,-0.144299303100741,
1.12357162229597));
#5207=CARTESIAN_POINT('Ctrl Pts',(0.006392292392153,-0.177024326825049,
1.12404235695137));
#5208=CARTESIAN_POINT('Ctrl Pts',(-0.0383992541984087,-0.227269801620063,
1.12335509974011));
#5209=CARTESIAN_POINT('Ctrl Pts',(-0.0680399972366993,-0.251265615809407,
1.12208997038458));
#5210=CARTESIAN_POINT('Ctrl Pts',(-0.117914228755037,-0.279889827963178,
1.1178344036749));
#5211=CARTESIAN_POINT('Ctrl Pts',(-0.14381238480104,-0.290879136862659,
1.11490049012186));
#5212=CARTESIAN_POINT('Ctrl Pts',(-0.19728546073067,-0.305251990234488,
1.10669035995599));
#5213=CARTESIAN_POINT('Ctrl Pts',(-0.224855950742601,-0.308638795020976,
1.10139101611326));
#5214=CARTESIAN_POINT('Ctrl Pts',(-0.275287440920027,-0.308638795020976,
1.0898803575765));
#5215=CARTESIAN_POINT('Ctrl Pts',(-0.302426893214945,-0.305251990234488,
1.08269251410343));
#5216=CARTESIAN_POINT('Ctrl Pts',(-0.35416671187353,-0.290879136862659,
1.06688848765783));
#5217=CARTESIAN_POINT('Ctrl Pts',(-0.3787731215897,-0.279889827963178,1.05829506364875));
#5218=CARTESIAN_POINT('Ctrl Pts',(-0.425554672694338,-0.251265615809407,
1.04048957871266));
#5219=CARTESIAN_POINT('Ctrl Pts',(-0.452808978448581,-0.227269801620063,
1.02876878445619));
#5220=CARTESIAN_POINT('Ctrl Pts',(-0.493462957200432,-0.177024326825049,
1.0099536580922));
#5221=CARTESIAN_POINT('Ctrl Pts',(-0.511762781179148,-0.14429930310074,
1.00061845128527));
#5222=CARTESIAN_POINT('Ctrl Pts',(-0.529268075276157,-0.0928409665394226,
0.991396466802468));
#5223=CARTESIAN_POINT('Ctrl Pts',(-0.533501897135713,-0.0762225747374254,
0.989110885965947));
#5224=CARTESIAN_POINT('Ctrl Pts',(-0.536443649899848,-0.0595300000000001,
0.987512846410683));
#5225=CARTESIAN_POINT('',(-0.843383895613249,-0.05953,0.742736168477219));
#5226=CARTESIAN_POINT('Origin',(0.,-0.05953,0.));
#5227=CARTESIAN_POINT('',(-1.10653577764992,-0.05953,0.196295654879792));
#5228=CARTESIAN_POINT('Ctrl Pts',(-0.843383895613249,-0.0595300000000001,
0.742736168477219));
#5229=CARTESIAN_POINT('Ctrl Pts',(-0.84559647055299,-0.0762225747374255,
0.740223768851062));
#5230=CARTESIAN_POINT('Ctrl Pts',(-0.848766861100456,-0.0928409665394227,
0.736604687327351));
#5231=CARTESIAN_POINT('Ctrl Pts',(-0.861652925570091,-0.144299303100741,
0.721590372101268));
#5232=CARTESIAN_POINT('Ctrl Pts',(-0.87482617317514,-0.177024326825049,
0.705826641853758));
#5233=CARTESIAN_POINT('Ctrl Pts',(-0.902215926359523,-0.227269801620063,
0.670378702718353));
#5234=CARTESIAN_POINT('Ctrl Pts',(-0.919707509403859,-0.251265615809407,
0.646415841396062));
#5235=CARTESIAN_POINT('Ctrl Pts',(-0.947476448101718,-0.279889827963178,
0.604769294586516));
#5236=CARTESIAN_POINT('Ctrl Pts',(-0.961329858300736,-0.290879136862659,
0.582692035672022));
#5237=CARTESIAN_POINT('Ctrl Pts',(-0.988250837578047,-0.305251990234488,
0.535766169015486));
#5238=CARTESIAN_POINT('Ctrl Pts',(-1.00129756308006,-0.308638795020976,
0.510906605094603));
#5239=CARTESIAN_POINT('Ctrl Pts',(-1.02374168767024,-0.308638795020976,
0.46430090015576));
#5240=CARTESIAN_POINT('Ctrl Pts',(-1.03504317708586,-0.305251990234488,
0.438600874831839));
#5241=CARTESIAN_POINT('Ctrl Pts',(-1.05494634094458,-0.290879136862659,
0.388295406390235));
#5242=CARTESIAN_POINT('Ctrl Pts',(-1.06356957703048,-0.279889827963178,
0.363699428370917));
#5243=CARTESIAN_POINT('Ctrl Pts',(-1.0788165083757,-0.251265615809407,0.316022600643821));
#5244=CARTESIAN_POINT('Ctrl Pts',(-1.08664560412098,-0.227269801620063,
0.287406530683752));
#5245=CARTESIAN_POINT('Ctrl Pts',(-1.09728268713976,-0.177024326825049,
0.243890930799337));
#5246=CARTESIAN_POINT('Ctrl Pts',(-1.10139388218929,-0.144299303100741,
0.22376314604679));
#5247=CARTESIAN_POINT('Ctrl Pts',(-1.10509821673782,-0.0928409665394227,
0.204327142733961));
#5248=CARTESIAN_POINT('Ctrl Pts',(-1.10595102243643,-0.0762225747374254,
0.199591971170104));
#5249=CARTESIAN_POINT('Ctrl Pts',(-1.10653577764992,-0.0595300000000001,
0.196295654879792));
#5250=CARTESIAN_POINT('',(-1.123812,-0.05953,1.37627276864339E-16));
#5251=CARTESIAN_POINT('Origin',(0.,-0.05953,0.));
#5252=CARTESIAN_POINT('',(-1.123812,-0.35718,1.37627276864339E-16));
#5253=CARTESIAN_POINT('',(-1.123812,-0.208355,1.37627276864339E-16));
#5254=CARTESIAN_POINT('Origin',(0.,-0.35718,0.));
#5255=CARTESIAN_POINT('',(-1.10653577764992,-0.05953,-0.196295654879793));
#5256=CARTESIAN_POINT('Origin',(0.,-0.05953,0.));
#5257=CARTESIAN_POINT('',(-0.843383895613249,-0.05953,-0.742736168477219));
#5258=CARTESIAN_POINT('Ctrl Pts',(-1.10653577764992,-0.0595300000000001,
-0.196295654879792));
#5259=CARTESIAN_POINT('Ctrl Pts',(-1.10595102243643,-0.0762225747374255,
-0.199591971170104));
#5260=CARTESIAN_POINT('Ctrl Pts',(-1.10509821673782,-0.0928409665394228,
-0.204327142733962));
#5261=CARTESIAN_POINT('Ctrl Pts',(-1.10139388218929,-0.144299303100741,
-0.22376314604679));
#5262=CARTESIAN_POINT('Ctrl Pts',(-1.09728268713976,-0.177024326825049,
-0.243890930799338));
#5263=CARTESIAN_POINT('Ctrl Pts',(-1.08664560412098,-0.227269801620063,
-0.287406530683753));
#5264=CARTESIAN_POINT('Ctrl Pts',(-1.0788165083757,-0.251265615809407,-0.316022600643821));
#5265=CARTESIAN_POINT('Ctrl Pts',(-1.06356957703048,-0.279889827963178,
-0.363699428370918));
#5266=CARTESIAN_POINT('Ctrl Pts',(-1.05494634094458,-0.290879136862659,
-0.388295406390235));
#5267=CARTESIAN_POINT('Ctrl Pts',(-1.03504317708586,-0.305251990234488,
-0.438600874831839));
#5268=CARTESIAN_POINT('Ctrl Pts',(-1.02374168767024,-0.308638795020976,
-0.46430090015576));
#5269=CARTESIAN_POINT('Ctrl Pts',(-1.00129756308006,-0.308638795020976,
-0.510906605094603));
#5270=CARTESIAN_POINT('Ctrl Pts',(-0.988250837578047,-0.305251990234488,
-0.535766169015486));
#5271=CARTESIAN_POINT('Ctrl Pts',(-0.961329858300736,-0.290879136862659,
-0.582692035672022));
#5272=CARTESIAN_POINT('Ctrl Pts',(-0.947476448101718,-0.279889827963178,
-0.604769294586516));
#5273=CARTESIAN_POINT('Ctrl Pts',(-0.919707509403859,-0.251265615809407,
-0.646415841396062));
#5274=CARTESIAN_POINT('Ctrl Pts',(-0.902215926359523,-0.227269801620064,
-0.670378702718353));
#5275=CARTESIAN_POINT('Ctrl Pts',(-0.87482617317514,-0.177024326825049,
-0.705826641853758));
#5276=CARTESIAN_POINT('Ctrl Pts',(-0.861652925570091,-0.144299303100741,
-0.721590372101268));
#5277=CARTESIAN_POINT('Ctrl Pts',(-0.848766861100456,-0.0928409665394229,
-0.736604687327351));
#5278=CARTESIAN_POINT('Ctrl Pts',(-0.84559647055299,-0.0762225747374255,
-0.740223768851063));
#5279=CARTESIAN_POINT('Ctrl Pts',(-0.843383895613249,-0.0595300000000001,
-0.742736168477219));
#5280=CARTESIAN_POINT('',(-0.536443649899847,-0.05953,-0.987512846410683));
#5281=CARTESIAN_POINT('Origin',(0.,-0.05953,0.));
#5282=CARTESIAN_POINT('',(0.0548532617164172,-0.05953,-1.12247250791415));
#5283=CARTESIAN_POINT('Ctrl Pts',(-0.536443649899848,-0.0595300000000001,
-0.987512846410683));
#5284=CARTESIAN_POINT('Ctrl Pts',(-0.533501897135712,-0.0762225747374254,
-0.989110885965947));
#5285=CARTESIAN_POINT('Ctrl Pts',(-0.529268075276156,-0.0928409665394227,
-0.991396466802469));
#5286=CARTESIAN_POINT('Ctrl Pts',(-0.511762781179147,-0.144299303100741,
-1.00061845128527));
#5287=CARTESIAN_POINT('Ctrl Pts',(-0.493462957200432,-0.177024326825049,
-1.0099536580922));
#5288=CARTESIAN_POINT('Ctrl Pts',(-0.45280897844858,-0.227269801620063,
-1.02876878445619));
#5289=CARTESIAN_POINT('Ctrl Pts',(-0.425554672694337,-0.251265615809407,
-1.04048957871266));
#5290=CARTESIAN_POINT('Ctrl Pts',(-0.3787731215897,-0.279889827963178,-1.05829506364875));
#5291=CARTESIAN_POINT('Ctrl Pts',(-0.354166711873529,-0.290879136862659,
-1.06688848765783));
#5292=CARTESIAN_POINT('Ctrl Pts',(-0.302426893214944,-0.305251990234488,
-1.08269251410343));
#5293=CARTESIAN_POINT('Ctrl Pts',(-0.275287440920027,-0.308638795020976,
-1.0898803575765));
#5294=CARTESIAN_POINT('Ctrl Pts',(-0.224855950742601,-0.308638795020976,
-1.10139101611326));
#5295=CARTESIAN_POINT('Ctrl Pts',(-0.19728546073067,-0.305251990234488,
-1.10669035995599));
#5296=CARTESIAN_POINT('Ctrl Pts',(-0.143812384801039,-0.290879136862659,
-1.11490049012186));
#5297=CARTESIAN_POINT('Ctrl Pts',(-0.117914228755037,-0.279889827963178,
-1.1178344036749));
#5298=CARTESIAN_POINT('Ctrl Pts',(-0.0680399972366989,-0.251265615809407,
-1.12208997038458));
#5299=CARTESIAN_POINT('Ctrl Pts',(-0.0383992541984084,-0.227269801620063,
-1.12335509974011));
#5300=CARTESIAN_POINT('Ctrl Pts',(0.00639229239215326,-0.177024326825049,
-1.12404235695137));
#5301=CARTESIAN_POINT('Ctrl Pts',(0.0269302585198977,-0.144299303100741,
-1.12357162229597));
#5302=CARTESIAN_POINT('Ctrl Pts',(0.04670325263426,-0.0928409665394228,
-1.12285816383385));
#5303=CARTESIAN_POINT('Ctrl Pts',(0.0515094706813703,-0.0762225747374255,
-1.12263591311425));
#5304=CARTESIAN_POINT('Ctrl Pts',(0.0548532617164176,-0.0595300000000001,
-1.12247250791414));
#5305=CARTESIAN_POINT('',(0.437601487681057,-0.05953,-1.03511272300331));
#5306=CARTESIAN_POINT('Origin',(0.,-0.05953,0.));
#5307=CARTESIAN_POINT('',(0.911784794170997,-0.05953,-0.656964154625313));
#5308=CARTESIAN_POINT('Ctrl Pts',(0.437601487681056,-0.0595300000000001,
-1.03511272300331));
#5309=CARTESIAN_POINT('Ctrl Pts',(0.440685038163619,-0.0762225747374255,
-1.03380912944435));
#5310=CARTESIAN_POINT('Ctrl Pts',(0.445111721969657,-0.0928409665394228,
-1.03192403056628));
#5311=CARTESIAN_POINT('Ctrl Pts',(0.463236132117164,-0.144299303100741,
-1.0239876538093));
#5312=CARTESIAN_POINT('Ctrl Pts',(0.481944444320713,-0.177024326825049,
-1.01550068154148));
#5313=CARTESIAN_POINT('Ctrl Pts',(0.522002043615455,-0.227269801620064,
-0.995447160474328));
#5314=CARTESIAN_POINT('Ctrl Pts',(0.548158511259203,-0.251265615809407,
-0.981446681891443));
#5315=CARTESIAN_POINT('Ctrl Pts',(0.591247219971725,-0.279889827963178,
-0.955972930713954));
#5316=CARTESIAN_POINT('Ctrl Pts',(0.613307674922609,-0.290879136862659,
-0.942092777160053));
#5317=CARTESIAN_POINT('Ctrl Pts',(0.657923009631182,-0.305251990234487,
-0.91149460735272));
#5318=CARTESIAN_POINT('Ctrl Pts',(0.680463863683393,-0.308638795020976,
-0.894757676234429));
#5319=CARTESIAN_POINT('Ctrl Pts',(0.720906778729542,-0.308638795020976,
-0.862505527716294));
#5320=CARTESIAN_POINT('Ctrl Pts',(0.742239891936899,-0.305251990234488,
-0.844254137480381));
#5321=CARTESIAN_POINT('Ctrl Pts',(0.781998747691872,-0.290879136862659,
-0.80756613568454));
#5322=CARTESIAN_POINT('Ctrl Pts',(0.800439809856112,-0.279889827963178,
-0.789147407129765));
#5323=CARTESIAN_POINT('Ctrl Pts',(0.834863020612702,-0.251265615809407,
-0.752807465209441));
#5324=CARTESIAN_POINT('Ctrl Pts',(0.854332839576145,-0.227269801620064,
-0.73042219438957));
#5325=CARTESIAN_POINT('Ctrl Pts',(0.882797231409153,-0.177024326825049,
-0.695831250979106));
#5326=CARTESIAN_POINT('Ctrl Pts',(0.895234408667242,-0.144299303100741,
-0.679480524217551));
#5327=CARTESIAN_POINT('Ctrl Pts',(0.907004864562642,-0.0928409665394228,
-0.663576540841106));
#5328=CARTESIAN_POINT('Ctrl Pts',(0.909827729890942,-0.0762225747374256,
-0.659680317203144));
#5329=CARTESIAN_POINT('Ctrl Pts',(0.911784794170998,-0.0595300000000001,
-0.656964154625312));
#5330=CARTESIAN_POINT('',(1.08212377959455,-0.05953,-0.303251606722892));
#5331=CARTESIAN_POINT('Origin',(0.,-0.05953,0.));
#5332=CARTESIAN_POINT('',(1.08212377959455,-0.05953,0.303251606722892));
#5333=CARTESIAN_POINT('Ctrl Pts',(1.08212377959455,-0.0595300000000001,
-0.303251606722892));
#5334=CARTESIAN_POINT('Ctrl Pts',(1.0830271513892,-0.0762225747374255,-0.300028012588062));
#5335=CARTESIAN_POINT('Ctrl Pts',(1.08431331394788,-0.0928409665394228,
-0.2953917518996));
#5336=CARTESIAN_POINT('Ctrl Pts',(1.08940878963422,-0.144299303100741,-0.276273267473431));
#5337=CARTESIAN_POINT('Ctrl Pts',(1.09443784939331,-0.177024326825049,-0.256354979351213));
#5338=CARTESIAN_POINT('Ctrl Pts',(1.10373487993589,-0.227269801620064,-0.212533521233765));
#5339=CARTESIAN_POINT('Ctrl Pts',(1.10909715583869,-0.251265615809407,-0.183354415742157));
#5340=CARTESIAN_POINT('Ctrl Pts',(1.1160463456491,-0.279889827963178,-0.133783682657561));
#5341=CARTESIAN_POINT('Ctrl Pts',(1.11894887330541,-0.290879136862659,-0.107881990270302));
#5342=CARTESIAN_POINT('Ctrl Pts',(1.12284346704144,-0.305251990234488,-0.0539226701638766));
#5343=CARTESIAN_POINT('Ctrl Pts',(1.123812,-0.308638795020976,-0.025864214957475));
#5344=CARTESIAN_POINT('Ctrl Pts',(1.123812,-0.308638795020976,0.025864214957475));
#5345=CARTESIAN_POINT('Ctrl Pts',(1.12284346704144,-0.305251990234488,0.0539226701638766));
#5346=CARTESIAN_POINT('Ctrl Pts',(1.11894887330541,-0.290879136862659,0.107881990270302));
#5347=CARTESIAN_POINT('Ctrl Pts',(1.1160463456491,-0.279889827963178,0.133783682657561));
#5348=CARTESIAN_POINT('Ctrl Pts',(1.10909715583869,-0.251265615809407,0.183354415742157));
#5349=CARTESIAN_POINT('Ctrl Pts',(1.10373487993589,-0.227269801620064,0.212533521233765));
#5350=CARTESIAN_POINT('Ctrl Pts',(1.09443784939331,-0.177024326825049,0.256354979351213));
#5351=CARTESIAN_POINT('Ctrl Pts',(1.08940878963422,-0.144299303100741,0.276273267473431));
#5352=CARTESIAN_POINT('Ctrl Pts',(1.08431331394788,-0.0928409665394228,
0.2953917518996));
#5353=CARTESIAN_POINT('Ctrl Pts',(1.0830271513892,-0.0762225747374255,0.300028012588062));
#5354=CARTESIAN_POINT('Ctrl Pts',(1.08212377959455,-0.0595300000000001,
0.303251606722892));
#5355=CARTESIAN_POINT('Origin',(0.,-0.05953,0.));
#5356=CARTESIAN_POINT('Origin',(0.,-0.05953,0.));
#5357=CARTESIAN_POINT('',(0.0589974094846122,-0.05953,1.07456964270265));
#5358=CARTESIAN_POINT('Origin',(0.,-0.05953,0.));
#5359=CARTESIAN_POINT('Origin',(-0.244773027351946,-0.05953,1.07242070340001));
#5360=CARTESIAN_POINT('Origin',(-0.244773027351946,0.,1.07242070340001));
#5361=CARTESIAN_POINT('',(-0.519393123750572,-0.05953,0.942555777842682));
#5362=CARTESIAN_POINT('Ctrl Pts',(-0.519393123750572,-0.05953,0.942555777842682));
#5363=CARTESIAN_POINT('Ctrl Pts',(-0.513714466572041,-0.0925528133349865,
0.945684988399766));
#5364=CARTESIAN_POINT('Ctrl Pts',(-0.503136848051455,-0.124911173756694,
0.951483858396181));
#5365=CARTESIAN_POINT('Ctrl Pts',(-0.47593627990192,-0.177924977804098,
0.965323333309091));
#5366=CARTESIAN_POINT('Ctrl Pts',(-0.460931856495794,-0.199697230012983,
0.972669835243841));
#5367=CARTESIAN_POINT('Ctrl Pts',(-0.426157505475872,-0.237895043532788,
0.988400002689705));
#5368=CARTESIAN_POINT('Ctrl Pts',(-0.406380688682952,-0.254319232363049,
0.996771768218699));
#5369=CARTESIAN_POINT('Ctrl Pts',(-0.364750145543744,-0.28018331644634,
1.01272583306292));
#5370=CARTESIAN_POINT('Ctrl Pts',(-0.340838910881557,-0.29104845371857,
1.02112815447116));
#5371=CARTESIAN_POINT('Ctrl Pts',(-0.290495481564827,-0.30527573347708,
1.036574285215));
#5372=CARTESIAN_POINT('Ctrl Pts',(-0.264056468041074,-0.308638795020976,
1.04359501395068));
#5373=CARTESIAN_POINT('Ctrl Pts',(-0.214892249704082,-0.308638795020976,
1.05481642595959));
#5374=CARTESIAN_POINT('Ctrl Pts',(-0.188025341585962,-0.30527573347708,
1.05996242598502));
#5375=CARTESIAN_POINT('Ctrl Pts',(-0.135965654106109,-0.29104845371857,
1.06788913840721));
#5376=CARTESIAN_POINT('Ctrl Pts',(-0.110776745452494,-0.28018331644634,
1.07069360430242));
#5377=CARTESIAN_POINT('Ctrl Pts',(-0.0663467128214646,-0.254319232363049,
1.07438230428002));
#5378=CARTESIAN_POINT('Ctrl Pts',(-0.0448960436540983,-0.237895043532788,
1.07542044338697));
#5379=CARTESIAN_POINT('Ctrl Pts',(-0.00674037211528124,-0.199697230012983,
1.07633607767727));
#5380=CARTESIAN_POINT('Ctrl Pts',(0.00996567398334777,-0.177924977804098,
1.07622728347683));
#5381=CARTESIAN_POINT('Ctrl Pts',(0.0404772621979741,-0.124911173756694,
1.07556023164702));
#5382=CARTESIAN_POINT('Ctrl Pts',(0.0525234025782719,-0.0925528133349865,
1.07492508698591));
#5383=CARTESIAN_POINT('Ctrl Pts',(0.0589974094846124,-0.05953,1.07456964270265));
#5384=CARTESIAN_POINT('Origin',(-0.244773027351946,-0.05953,1.07242070340001));
#5385=CARTESIAN_POINT('Origin',(0.,-0.05953,0.));
#5386=CARTESIAN_POINT('',(-0.803348093619616,-0.05953,0.716109245731214));
#5387=CARTESIAN_POINT('Origin',(0.,-0.05953,0.));
#5388=CARTESIAN_POINT('Origin',(-0.991065754692661,-0.05953,0.477272113029314));
#5389=CARTESIAN_POINT('Origin',(-0.991065754692661,0.,0.477272113029314));
#5390=CARTESIAN_POINT('',(-1.06075609691358,-0.05953,0.181596019242328));
#5391=CARTESIAN_POINT('Ctrl Pts',(-1.06075609691358,-0.05953,0.181596019242328));
#5392=CARTESIAN_POINT('Ctrl Pts',(-1.05966202740332,-0.0925528133349865,
0.187986803072856));
#5393=CARTESIAN_POINT('Ctrl Pts',(-1.05760072925372,-0.124911173756694,
0.199872254546857));
#5394=CARTESIAN_POINT('Ctrl Pts',(-1.05146158959546,-0.177924977804098,
0.22976728653846));
#5395=CARTESIAN_POINT('Ctrl Pts',(-1.04785021111757,-0.199697230012983,
0.246078686169301));
#5396=CARTESIAN_POINT('Ctrl Pts',(-1.03846709802406,-0.237895043532788,
0.283073967563097));
#5397=CARTESIAN_POINT('Ctrl Pts',(-1.03268176429485,-0.254319232363049,
0.303755815985685));
#5398=CARTESIAN_POINT('Ctrl Pts',(-1.01919893537026,-0.28018331644634,0.346251081972725));
#5399=CARTESIAN_POINT('Ctrl Pts',(-1.01085972381132,-0.29104845371857,0.370184399726282));
#5400=CARTESIAN_POINT('Ctrl Pts',(-0.99154738033959,-0.30527573347708,0.419174982698463));
#5401=CARTESIAN_POINT('Ctrl Pts',(-0.980551951791748,-0.308638795020976,
0.444223188605045));
#5402=CARTESIAN_POINT('Ctrl Pts',(-0.958671816228589,-0.308638795020976,
0.489657758261848));
#5403=CARTESIAN_POINT('Ctrl Pts',(-0.945943877838127,-0.30527573347708,
0.51387163140139));
#5404=CARTESIAN_POINT('Ctrl Pts',(-0.91968254693063,-0.29104845371857,0.559515758398093));
#5405=CARTESIAN_POINT('Ctrl Pts',(-0.906170138993533,-0.28018331644634,
0.580957796077825));
#5406=CARTESIAN_POINT('Ctrl Pts',(-0.8813524085237,-0.254319232363049,0.617994461173994));
#5407=CARTESIAN_POINT('Ctrl Pts',(-0.868789784891799,-0.237895043532788,
0.635412538795143));
#5408=CARTESIAN_POINT('Ctrl Pts',(-0.845715984518854,-0.199697230012983,
0.66581473268113));
#5409=CARTESIAN_POINT('Ctrl Pts',(-0.835214876415962,-0.177924977804098,
0.678808213394124));
#5410=CARTESIAN_POINT('Ctrl Pts',(-0.815669690204649,-0.124911173756694,
0.702247233627224));
#5411=CARTESIAN_POINT('Ctrl Pts',(-0.807662468433796,-0.0925528133349865,
0.711269279199861));
#5412=CARTESIAN_POINT('Ctrl Pts',(-0.803348093619616,-0.05953,0.716109245731214));
#5413=CARTESIAN_POINT('Origin',(-0.991065754692661,-0.05953,0.477272113029314));
#5414=CARTESIAN_POINT('Origin',(0.,-0.05953,0.));
#5415=CARTESIAN_POINT('',(-1.076188,-0.05953,1.31795018948079E-16));
#5416=CARTESIAN_POINT('Origin',(0.,-0.05953,0.));
#5417=CARTESIAN_POINT('',(-1.06075609691358,-0.05953,-0.181596019242328));
#5418=CARTESIAN_POINT('Origin',(0.,-0.05953,0.));
#5419=CARTESIAN_POINT('Origin',(-0.991065754692661,-0.05953,-0.477272113029314));
#5420=CARTESIAN_POINT('Origin',(-0.991065754692661,0.,-0.477272113029314));
#5421=CARTESIAN_POINT('',(-0.803348093619616,-0.05953,-0.716109245731215));
#5422=CARTESIAN_POINT('Ctrl Pts',(-0.803348093619616,-0.05953,-0.716109245731215));
#5423=CARTESIAN_POINT('Ctrl Pts',(-0.807662468433795,-0.0925528133349865,
-0.711269279199862));
#5424=CARTESIAN_POINT('Ctrl Pts',(-0.815669690204649,-0.124911173756694,
-0.702247233627224));
#5425=CARTESIAN_POINT('Ctrl Pts',(-0.835214876415962,-0.177924977804098,
-0.678808213394124));
#5426=CARTESIAN_POINT('Ctrl Pts',(-0.845715984518854,-0.199697230012983,
-0.66581473268113));
#5427=CARTESIAN_POINT('Ctrl Pts',(-0.868789784891799,-0.237895043532788,
-0.635412538795143));
#5428=CARTESIAN_POINT('Ctrl Pts',(-0.8813524085237,-0.254319232363049,-0.617994461173994));
#5429=CARTESIAN_POINT('Ctrl Pts',(-0.906170138993533,-0.28018331644634,
-0.580957796077826));
#5430=CARTESIAN_POINT('Ctrl Pts',(-0.91968254693063,-0.29104845371857,-0.559515758398093));
#5431=CARTESIAN_POINT('Ctrl Pts',(-0.945943877838127,-0.30527573347708,
-0.51387163140139));
#5432=CARTESIAN_POINT('Ctrl Pts',(-0.958671816228589,-0.308638795020976,
-0.489657758261848));
#5433=CARTESIAN_POINT('Ctrl Pts',(-0.980551951791748,-0.308638795020976,
-0.444223188605045));
#5434=CARTESIAN_POINT('Ctrl Pts',(-0.99154738033959,-0.30527573347708,-0.419174982698463));
#5435=CARTESIAN_POINT('Ctrl Pts',(-1.01085972381132,-0.29104845371857,-0.370184399726282));
#5436=CARTESIAN_POINT('Ctrl Pts',(-1.01919893537026,-0.28018331644634,-0.346251081972725));
#5437=CARTESIAN_POINT('Ctrl Pts',(-1.03268176429485,-0.254319232363049,
-0.303755815985685));
#5438=CARTESIAN_POINT('Ctrl Pts',(-1.03846709802406,-0.237895043532788,
-0.283073967563097));
#5439=CARTESIAN_POINT('Ctrl Pts',(-1.04785021111757,-0.199697230012983,
-0.246078686169302));
#5440=CARTESIAN_POINT('Ctrl Pts',(-1.05146158959546,-0.177924977804098,
-0.229767286538461));
#5441=CARTESIAN_POINT('Ctrl Pts',(-1.05760072925372,-0.124911173756694,
-0.199872254546858));
#5442=CARTESIAN_POINT('Ctrl Pts',(-1.05966202740332,-0.0925528133349864,
-0.187986803072857));
#5443=CARTESIAN_POINT('Ctrl Pts',(-1.06075609691358,-0.05953,-0.181596019242328));
#5444=CARTESIAN_POINT('Origin',(-0.991065754692661,-0.05953,-0.477272113029314));
#5445=CARTESIAN_POINT('Origin',(0.,-0.05953,0.));
#5446=CARTESIAN_POINT('',(-0.519393123750572,-0.05953,-0.942555777842682));
#5447=CARTESIAN_POINT('Origin',(0.,-0.05953,0.));
#5448=CARTESIAN_POINT('Origin',(-0.244773027351946,-0.05953,-1.07242070340001));
#5449=CARTESIAN_POINT('Origin',(-0.244773027351946,0.,-1.07242070340001));
#5450=CARTESIAN_POINT('',(0.0589974094846125,-0.05953,-1.07456964270265));
#5451=CARTESIAN_POINT('Ctrl Pts',(0.0589974094846127,-0.05953,-1.07456964270265));
#5452=CARTESIAN_POINT('Ctrl Pts',(0.0525234025782722,-0.0925528133349865,
-1.07492508698591));
#5453=CARTESIAN_POINT('Ctrl Pts',(0.0404772621979744,-0.124911173756694,
-1.07556023164702));
#5454=CARTESIAN_POINT('Ctrl Pts',(0.0099656739833481,-0.177924977804098,
-1.07622728347683));
#5455=CARTESIAN_POINT('Ctrl Pts',(-0.00674037211528096,-0.199697230012983,
-1.07633607767727));
#5456=CARTESIAN_POINT('Ctrl Pts',(-0.044896043654098,-0.237895043532788,
-1.07542044338697));
#5457=CARTESIAN_POINT('Ctrl Pts',(-0.0663467128214644,-0.254319232363049,
-1.07438230428002));
#5458=CARTESIAN_POINT('Ctrl Pts',(-0.110776745452493,-0.28018331644634,
-1.07069360430242));
#5459=CARTESIAN_POINT('Ctrl Pts',(-0.135965654106109,-0.29104845371857,
-1.06788913840721));
#5460=CARTESIAN_POINT('Ctrl Pts',(-0.188025341585962,-0.30527573347708,
-1.05996242598502));
#5461=CARTESIAN_POINT('Ctrl Pts',(-0.214892249704082,-0.308638795020976,
-1.05481642595959));
#5462=CARTESIAN_POINT('Ctrl Pts',(-0.264056468041074,-0.308638795020976,
-1.04359501395068));
#5463=CARTESIAN_POINT('Ctrl Pts',(-0.290495481564827,-0.30527573347708,
-1.036574285215));
#5464=CARTESIAN_POINT('Ctrl Pts',(-0.340838910881557,-0.291048453718569,
-1.02112815447116));
#5465=CARTESIAN_POINT('Ctrl Pts',(-0.364750145543744,-0.28018331644634,
-1.01272583306292));
#5466=CARTESIAN_POINT('Ctrl Pts',(-0.406380688682952,-0.254319232363049,
-0.996771768218699));
#5467=CARTESIAN_POINT('Ctrl Pts',(-0.426157505475872,-0.237895043532788,
-0.988400002689705));
#5468=CARTESIAN_POINT('Ctrl Pts',(-0.460931856495794,-0.199697230012983,
-0.972669835243841));
#5469=CARTESIAN_POINT('Ctrl Pts',(-0.475936279901919,-0.177924977804098,
-0.965323333309091));
#5470=CARTESIAN_POINT('Ctrl Pts',(-0.503136848051454,-0.124911173756694,
-0.951483858396181));
#5471=CARTESIAN_POINT('Ctrl Pts',(-0.513714466572041,-0.0925528133349865,
-0.945684988399766));
#5472=CARTESIAN_POINT('Ctrl Pts',(-0.519393123750572,-0.05953,-0.942555777842682));
#5473=CARTESIAN_POINT('Origin',(-0.244773027351946,-0.05953,-1.07242070340001));
#5474=CARTESIAN_POINT('Origin',(0.,-0.05953,0.));
#5475=CARTESIAN_POINT('',(0.413083465285518,-0.05953,-0.993751811093549));
#5476=CARTESIAN_POINT('Origin',(0.,-0.05953,0.));
#5477=CARTESIAN_POINT('Origin',(0.685838782044607,-0.05953,-0.860014630714833));
#5478=CARTESIAN_POINT('Origin',(0.685838782044607,0.,-0.860014630714833));
#5479=CARTESIAN_POINT('',(0.876916659919095,-0.05953,-0.623857181492959));
#5480=CARTESIAN_POINT('Ctrl Pts',(0.876916659919095,-0.05953,-0.623857181492958));
#5481=CARTESIAN_POINT('Ctrl Pts',(0.873158080166742,-0.0925528133349865,
-0.62914037979579));
#5482=CARTESIAN_POINT('Ctrl Pts',(0.866144010579847,-0.124911173756694,
-0.638954437806245));
#5483=CARTESIAN_POINT('Ctrl Pts',(0.847641868610495,-0.177924977804098,
-0.663225258065736));
#5484=CARTESIAN_POINT('Ctrl Pts',(0.837310877969633,-0.199697230012983,
-0.676354402927683));
#5485=CARTESIAN_POINT('Ctrl Pts',(0.81280533416753,-0.237895043532788,-0.705614819529209));
#5486=CARTESIAN_POINT('Ctrl Pts',(0.798619410861634,-0.254319232363049,
-0.721738358858166));
#5487=CARTESIAN_POINT('Ctrl Pts',(0.768033796848072,-0.28018331644634,-0.754175290318038));
#5488=CARTESIAN_POINT('Ctrl Pts',(0.750136149454208,-0.29104845371857,-0.772120216227122));
#5489=CARTESIAN_POINT('Ctrl Pts',(0.711480111898423,-0.30527573347708,-0.807879894508811));
#5490=CARTESIAN_POINT('Ctrl Pts',(0.690705563850638,-0.308638795020976,
-0.825676810575913));
#5491=CARTESIAN_POINT('Ctrl Pts',(0.651278921914856,-0.308638795020976,
-0.857118508332695));
#5492=CARTESIAN_POINT('Ctrl Pts',(0.629305439856167,-0.30527573347708,-0.873412008702649));
#5493=CARTESIAN_POINT('Ctrl Pts',(0.585840553788742,-0.29104845371857,-0.903141581680914));
#5494=CARTESIAN_POINT('Ctrl Pts',(0.564362943424239,-0.28018331644634,-0.916597376014514));
#5495=CARTESIAN_POINT('Ctrl Pts',(0.525933334162556,-0.254319232363049,
-0.939198248544427));
#5496=CARTESIAN_POINT('Ctrl Pts',(0.507057380724533,-0.237895043532788,
-0.949440676105255));
#5497=CARTESIAN_POINT('Ctrl Pts',(0.473077587363686,-0.199697230012983,
-0.966820759530997));
#5498=CARTESIAN_POINT('Ctrl Pts',(0.457978755888596,-0.177924977804098,
-0.973971221090534));
#5499=CARTESIAN_POINT('Ctrl Pts',(0.430199341854858,-0.124911173756694,
-0.986608710139579));
#5500=CARTESIAN_POINT('Ctrl Pts',(0.419070565453384,-0.0925528133349865,
-0.991263089003441));
#5501=CARTESIAN_POINT('Ctrl Pts',(0.413083465285518,-0.05953,-0.993751811093549));
#5502=CARTESIAN_POINT('Origin',(0.685838782044607,-0.05953,-0.860014630714833));
#5503=CARTESIAN_POINT('Origin',(0.,-0.208355,0.));
#5504=CARTESIAN_POINT('',(-1.076188,-0.35718,1.31795018948079E-16));
#5505=CARTESIAN_POINT('Origin',(0.,-0.35718,0.));
#5506=CARTESIAN_POINT('',(-1.076188,-0.208355,1.31795018948079E-16));
#5507=CARTESIAN_POINT('',(1.03449977959455,-0.05953,0.296632461748266));
#5508=CARTESIAN_POINT('Origin',(0.,-0.05953,0.));
#5509=CARTESIAN_POINT('',(1.03449977959455,-0.05953,-0.296632461748266));
#5510=CARTESIAN_POINT('Ctrl Pts',(1.03449977959455,-0.05953,0.296632461748267));
#5511=CARTESIAN_POINT('Ctrl Pts',(1.03628691421076,-0.0925528133349865,
0.290399865505497));
#5512=CARTESIAN_POINT('Ctrl Pts',(1.03958665287714,-0.124911173756694,0.278797079997872));
#5513=CARTESIAN_POINT('Ctrl Pts',(1.0470264474309,-0.177924977804098,0.249198913998601));
#5514=CARTESIAN_POINT('Ctrl Pts',(1.05084995891418,-0.199697230012983,0.232935932341942));
#5515=CARTESIAN_POINT('Ctrl Pts',(1.05844771715377,-0.237895043532788,0.195533155353269));
#5516=CARTESIAN_POINT('Ctrl Pts',(1.06220882929878,-0.254319232363049,0.17438929156337));
#5517=CARTESIAN_POINT('Ctrl Pts',(1.06849922508772,-0.28018331644634,0.130252399648131));
#5518=CARTESIAN_POINT('Ctrl Pts',(1.07137013248666,-0.29104845371857,0.105070977154072));
#5519=CARTESIAN_POINT('Ctrl Pts',(1.07522652957392,-0.30527573347708,0.0525526752791107));
#5520=CARTESIAN_POINT('Ctrl Pts',(1.076188,-0.308638795020976,0.025214283908933));
#5521=CARTESIAN_POINT('Ctrl Pts',(1.076188,-0.308638795020976,-0.025214283908933));
#5522=CARTESIAN_POINT('Ctrl Pts',(1.07522652957392,-0.30527573347708,-0.0525526752791107));
#5523=CARTESIAN_POINT('Ctrl Pts',(1.07137013248666,-0.29104845371857,-0.105070977154072));
#5524=CARTESIAN_POINT('Ctrl Pts',(1.06849922508772,-0.28018331644634,-0.130252399648131));
#5525=CARTESIAN_POINT('Ctrl Pts',(1.06220882929878,-0.254319232363049,-0.17438929156337));
#5526=CARTESIAN_POINT('Ctrl Pts',(1.05844771715377,-0.237895043532788,-0.195533155353269));
#5527=CARTESIAN_POINT('Ctrl Pts',(1.05084995891418,-0.199697230012983,-0.232935932341942));
#5528=CARTESIAN_POINT('Ctrl Pts',(1.0470264474309,-0.177924977804098,-0.249198913998601));
#5529=CARTESIAN_POINT('Ctrl Pts',(1.03958665287714,-0.124911173756694,-0.278797079997872));
#5530=CARTESIAN_POINT('Ctrl Pts',(1.03628691421076,-0.0925528133349865,
-0.290399865505497));
#5531=CARTESIAN_POINT('Ctrl Pts',(1.03449977959455,-0.05953,-0.296632461748267));
#5532=CARTESIAN_POINT('Origin',(0.,-0.05953,0.));
#5533=CARTESIAN_POINT('Origin',(0.,-0.05953,0.));
#5534=CARTESIAN_POINT('Origin',(1.1,-0.05953,0.));
#5535=CARTESIAN_POINT('Origin',(1.1,0.,0.));
#5536=CARTESIAN_POINT('Origin',(1.1,-0.05953,0.));
#5537=CARTESIAN_POINT('Origin',(0.,-0.35718,0.));
#5538=CARTESIAN_POINT('Origin',(0.,-0.05953,0.));
#5705=UNCERTAINTY_MEASURE_WITH_UNIT(LENGTH_MEASURE(0.001),#5735,
'DISTANCE_ACCURACY_VALUE',
'Maximum model space distance between geometric entities at asserted c
onnectivities');
#5711=UNCERTAINTY_MEASURE_WITH_UNIT(LENGTH_MEASURE(0.001),#5735,
'DISTANCE_ACCURACY_VALUE',
'Maximum model space distance between geometric entities at asserted c
onnectivities');
#5728=(
GEOMETRIC_REPRESENTATION_CONTEXT(3)
GLOBAL_UNCERTAINTY_ASSIGNED_CONTEXT((#5705))
GLOBAL_UNIT_ASSIGNED_CONTEXT((#5735,#5737,#5738))
REPRESENTATION_CONTEXT('','3D')
);
#5734=(
GEOMETRIC_REPRESENTATION_CONTEXT(3)
GLOBAL_UNCERTAINTY_ASSIGNED_CONTEXT((#5711))
GLOBAL_UNIT_ASSIGNED_CONTEXT((#5735,#5737,#5738))
REPRESENTATION_CONTEXT('','3D')
);
#5735=(
LENGTH_UNIT()
NAMED_UNIT(*)
SI_UNIT(.CENTI.,.METRE.)
);
#5737=(
NAMED_UNIT(*)
PLANE_ANGLE_UNIT()
SI_UNIT($,.RADIAN.)
);
#5738=(
NAMED_UNIT(*)
SI_UNIT($,.STERADIAN.)
SOLID_ANGLE_UNIT()
);
#5755=SHAPE_DEFINITION_REPRESENTATION(#5787,#5824);
#5787=PRODUCT_DEFINITION_SHAPE('',$,#5847);
#5824=SHAPE_REPRESENTATION('',(#3443),#5728);
#5830=PRODUCT_DEFINITION_CONTEXT('part definition',#5898,'design');
#5847=PRODUCT_DEFINITION('Cage','Cage',#5869,#5830);
#5869=PRODUCT_DEFINITION_FORMATION('',$,#5916);
#5898=APPLICATION_CONTEXT(
'Core Data for Automotive Mechanical Design Process');
#5899=PRODUCT_CONTEXT('part definition',#5898,'mechanical');
#5916=PRODUCT('Cage','Cage','Cage',(#5899));
#5978=COLOUR_RGB('Grey',0.48,0.52,0.57);
#5979=FILL_AREA_STYLE_COLOUR('',#5978);
#5980=FILL_AREA_STYLE('',(#5979));
#5981=SURFACE_STYLE_FILL_AREA(#5980);
#5982=SURFACE_SIDE_STYLE('',(#5981));
#5983=SURFACE_STYLE_USAGE(.BOTH.,#5982);
#5984=PRESENTATION_STYLE_ASSIGNMENT((#5983));
ENDSEC;
END-ISO-10303-21;
